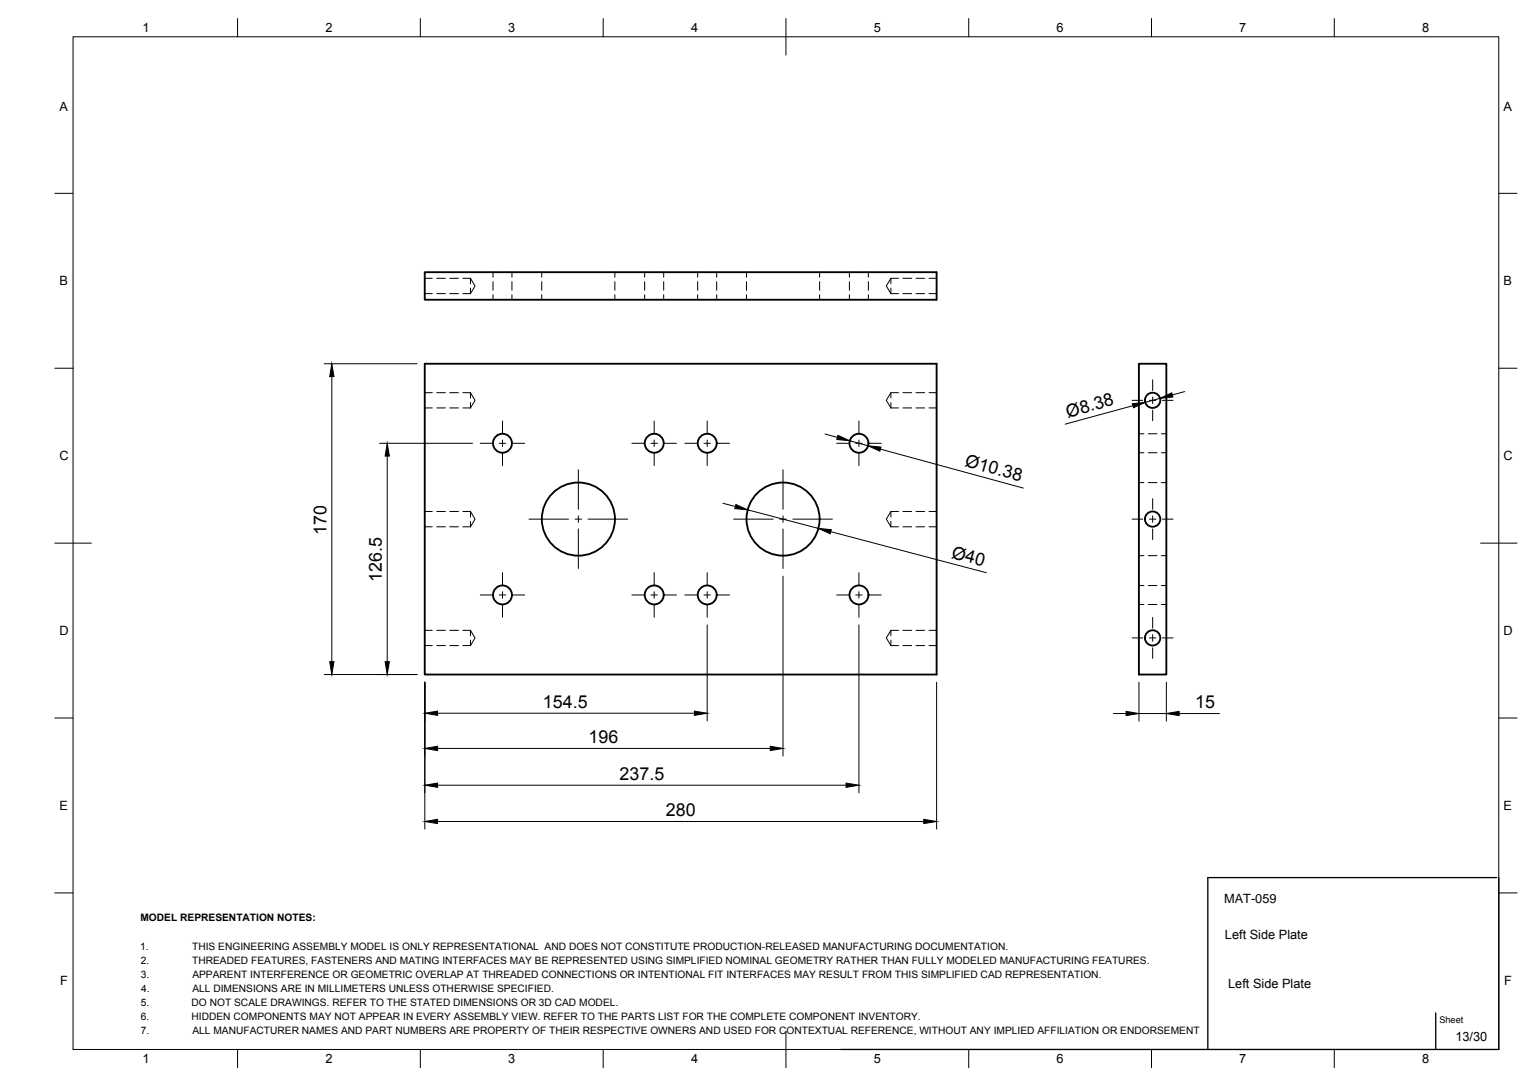
ISO-10303-21;
HEADER;
/* Generated by software containing ST-Developer
 * from STEP Tools, Inc. (www.steptools.com) 
 */

FILE_DESCRIPTION(
/* description */ ('', 'CAx-IF Rec.Pracs.---Representation and Presentation of Product Manufa
cturing Information (PMI)---4.0---2014-10-13'),
/* implementation_level */ '2;1');

FILE_NAME(
/* name */ 'Left Side Plate.step',
/* time_stamp */ '2026-10-28T23:00:48+01:00',
/* author */ (''),
/* organization */ (''),
/* preprocessor_version */ 'ST-DEVELOPER v20.2',
/* originating_system */ 'Autodesk Translation Framework v15.17.0.0',
/* authorisation */ '');

FILE_SCHEMA (('AP242_MANAGED_MODEL_BASED_3D_ENGINEERING_MIM_LF { 1 0 10303 442 2 1 4 }'));
ENDSEC;

DATA;
#10=MECHANICAL_DESIGN_GEOMETRIC_PRESENTATION_REPRESENTATION('',(#987),#61811);
#591=CONICAL_SURFACE('',#35772,2.094,1.02974425867665);
#592=CONICAL_SURFACE('',#35775,2.094,1.02974425867665);
#593=CONICAL_SURFACE('',#35778,2.094,1.02974425867665);
#594=CONICAL_SURFACE('',#35781,2.094,1.02974425867665);
#595=CONICAL_SURFACE('',#35784,2.094,1.02974425867665);
#596=CONICAL_SURFACE('',#35787,2.094,1.02974425867665);
#923=SHAPE_REPRESENTATION_RELATIONSHIP('SRR','None',#61982,#948);
#948=ADVANCED_BREP_SHAPE_REPRESENTATION('',(#1026),#61795);
#987=STYLED_ITEM('',(#62142),#1026);
#1026=MANIFOLD_SOLID_BREP('Body1',#33817);
#1327=CYLINDRICAL_SURFACE('',#35774,4.188);
#1328=CYLINDRICAL_SURFACE('',#35777,4.188);
#1329=CYLINDRICAL_SURFACE('',#35780,4.188);
#1330=CYLINDRICAL_SURFACE('',#35783,4.188);
#1331=CYLINDRICAL_SURFACE('',#35786,4.188);
#1332=CYLINDRICAL_SURFACE('',#35789,4.188);
#1333=CYLINDRICAL_SURFACE('',#35790,5.188);
#1334=CYLINDRICAL_SURFACE('',#35793,5.188);
#1335=CYLINDRICAL_SURFACE('',#35796,5.188);
#1336=CYLINDRICAL_SURFACE('',#35799,5.188);
#1337=CYLINDRICAL_SURFACE('',#35802,5.188);
#1338=CYLINDRICAL_SURFACE('',#35805,5.188);
#1339=CYLINDRICAL_SURFACE('',#35808,5.188);
#1340=CYLINDRICAL_SURFACE('',#35811,5.188);
#1341=CYLINDRICAL_SURFACE('',#35814,20.);
#1342=CYLINDRICAL_SURFACE('',#35817,20.);
#2042=FACE_BOUND('',#7145,.T.);
#2043=FACE_BOUND('',#7146,.T.);
#2044=FACE_BOUND('',#7147,.T.);
#2045=FACE_BOUND('',#7149,.T.);
#2046=FACE_BOUND('',#7150,.T.);
#2047=FACE_BOUND('',#7151,.T.);
#2048=FACE_BOUND('',#7176,.T.);
#2049=FACE_BOUND('',#7177,.T.);
#2050=FACE_BOUND('',#7178,.T.);
#2051=FACE_BOUND('',#7179,.T.);
#2052=FACE_BOUND('',#7180,.T.);
#2053=FACE_BOUND('',#7181,.T.);
#2054=FACE_BOUND('',#7182,.T.);
#2055=FACE_BOUND('',#7183,.T.);
#2056=FACE_BOUND('',#7184,.T.);
#2057=FACE_BOUND('',#7185,.T.);
#2058=FACE_BOUND('',#7188,.T.);
#2059=FACE_BOUND('',#7189,.T.);
#2060=FACE_BOUND('',#7190,.T.);
#2061=FACE_BOUND('',#7191,.T.);
#2062=FACE_BOUND('',#7192,.T.);
#2063=FACE_BOUND('',#7193,.T.);
#2064=FACE_BOUND('',#7194,.T.);
#2065=FACE_BOUND('',#7195,.T.);
#2066=FACE_BOUND('',#7196,.T.);
#2067=FACE_BOUND('',#7197,.T.);
#2952=CIRCLE('',#35764,4.188);
#2953=CIRCLE('',#35765,4.188);
#2954=CIRCLE('',#35766,4.188);
#2955=CIRCLE('',#35768,4.188);
#2956=CIRCLE('',#35769,4.188);
#2957=CIRCLE('',#35770,4.188);
#2958=CIRCLE('',#35773,4.188);
#2959=CIRCLE('',#35776,4.188);
#2960=CIRCLE('',#35779,4.188);
#2961=CIRCLE('',#35782,4.188);
#2962=CIRCLE('',#35785,4.188);
#2963=CIRCLE('',#35788,4.188);
#2964=CIRCLE('',#35791,5.188);
#2965=CIRCLE('',#35792,5.188);
#2966=CIRCLE('',#35794,5.188);
#2967=CIRCLE('',#35795,5.188);
#2968=CIRCLE('',#35797,5.188);
#2969=CIRCLE('',#35798,5.188);
#2970=CIRCLE('',#35800,5.188);
#2971=CIRCLE('',#35801,5.188);
#2972=CIRCLE('',#35803,5.188);
#2973=CIRCLE('',#35804,5.188);
#2974=CIRCLE('',#35806,5.188);
#2975=CIRCLE('',#35807,5.188);
#2976=CIRCLE('',#35809,5.188);
#2977=CIRCLE('',#35810,5.188);
#2978=CIRCLE('',#35812,5.188);
#2979=CIRCLE('',#35813,5.188);
#2980=CIRCLE('',#35815,20.);
#2981=CIRCLE('',#35816,20.);
#2982=CIRCLE('',#35818,20.);
#2983=CIRCLE('',#35819,20.);
#5102=FACE_OUTER_BOUND('',#7144,.T.);
#5103=FACE_OUTER_BOUND('',#7148,.T.);
#5104=FACE_OUTER_BOUND('',#7152,.T.);
#5105=FACE_OUTER_BOUND('',#7153,.T.);
#5106=FACE_OUTER_BOUND('',#7154,.T.);
#5107=FACE_OUTER_BOUND('',#7155,.T.);
#5108=FACE_OUTER_BOUND('',#7156,.T.);
#5109=FACE_OUTER_BOUND('',#7157,.T.);
#5110=FACE_OUTER_BOUND('',#7158,.T.);
#5111=FACE_OUTER_BOUND('',#7159,.T.);
#5112=FACE_OUTER_BOUND('',#7160,.T.);
#5113=FACE_OUTER_BOUND('',#7161,.T.);
#5114=FACE_OUTER_BOUND('',#7162,.T.);
#5115=FACE_OUTER_BOUND('',#7163,.T.);
#5116=FACE_OUTER_BOUND('',#7164,.T.);
#5117=FACE_OUTER_BOUND('',#7165,.T.);
#5118=FACE_OUTER_BOUND('',#7166,.T.);
#5119=FACE_OUTER_BOUND('',#7167,.T.);
#5120=FACE_OUTER_BOUND('',#7168,.T.);
#5121=FACE_OUTER_BOUND('',#7169,.T.);
#5122=FACE_OUTER_BOUND('',#7170,.T.);
#5123=FACE_OUTER_BOUND('',#7171,.T.);
#5124=FACE_OUTER_BOUND('',#7172,.T.);
#5125=FACE_OUTER_BOUND('',#7173,.T.);
#5126=FACE_OUTER_BOUND('',#7174,.T.);
#5127=FACE_OUTER_BOUND('',#7175,.T.);
#5128=FACE_OUTER_BOUND('',#7186,.T.);
#5129=FACE_OUTER_BOUND('',#7187,.T.);
#7144=EDGE_LOOP('',(#25798,#25799,#25800,#25801));
#7145=EDGE_LOOP('',(#25802));
#7146=EDGE_LOOP('',(#25803));
#7147=EDGE_LOOP('',(#25804));
#7148=EDGE_LOOP('',(#25805,#25806,#25807,#25808));
#7149=EDGE_LOOP('',(#25809));
#7150=EDGE_LOOP('',(#25810));
#7151=EDGE_LOOP('',(#25811));
#7152=EDGE_LOOP('',(#25812,#25813,#25814,#25815));
#7153=EDGE_LOOP('',(#25816,#25817,#25818));
#7154=EDGE_LOOP('',(#25819,#25820,#25821,#25822));
#7155=EDGE_LOOP('',(#25823,#25824,#25825));
#7156=EDGE_LOOP('',(#25826,#25827,#25828,#25829));
#7157=EDGE_LOOP('',(#25830,#25831,#25832));
#7158=EDGE_LOOP('',(#25833,#25834,#25835,#25836));
#7159=EDGE_LOOP('',(#25837,#25838,#25839));
#7160=EDGE_LOOP('',(#25840,#25841,#25842,#25843));
#7161=EDGE_LOOP('',(#25844,#25845,#25846));
#7162=EDGE_LOOP('',(#25847,#25848,#25849,#25850));
#7163=EDGE_LOOP('',(#25851,#25852,#25853));
#7164=EDGE_LOOP('',(#25854,#25855,#25856,#25857));
#7165=EDGE_LOOP('',(#25858,#25859,#25860,#25861));
#7166=EDGE_LOOP('',(#25862,#25863,#25864,#25865));
#7167=EDGE_LOOP('',(#25866,#25867,#25868,#25869));
#7168=EDGE_LOOP('',(#25870,#25871,#25872,#25873));
#7169=EDGE_LOOP('',(#25874,#25875,#25876,#25877));
#7170=EDGE_LOOP('',(#25878,#25879,#25880,#25881));
#7171=EDGE_LOOP('',(#25882,#25883,#25884,#25885));
#7172=EDGE_LOOP('',(#25886,#25887,#25888,#25889));
#7173=EDGE_LOOP('',(#25890,#25891,#25892,#25893));
#7174=EDGE_LOOP('',(#25894,#25895,#25896,#25897));
#7175=EDGE_LOOP('',(#25898,#25899,#25900,#25901));
#7176=EDGE_LOOP('',(#25902));
#7177=EDGE_LOOP('',(#25903));
#7178=EDGE_LOOP('',(#25904));
#7179=EDGE_LOOP('',(#25905));
#7180=EDGE_LOOP('',(#25906));
#7181=EDGE_LOOP('',(#25907));
#7182=EDGE_LOOP('',(#25908));
#7183=EDGE_LOOP('',(#25909));
#7184=EDGE_LOOP('',(#25910));
#7185=EDGE_LOOP('',(#25911));
#7186=EDGE_LOOP('',(#25912,#25913,#25914,#25915));
#7187=EDGE_LOOP('',(#25916,#25917,#25918,#25919));
#7188=EDGE_LOOP('',(#25920));
#7189=EDGE_LOOP('',(#25921));
#7190=EDGE_LOOP('',(#25922));
#7191=EDGE_LOOP('',(#25923));
#7192=EDGE_LOOP('',(#25924));
#7193=EDGE_LOOP('',(#25925));
#7194=EDGE_LOOP('',(#25926));
#7195=EDGE_LOOP('',(#25927));
#7196=EDGE_LOOP('',(#25928));
#7197=EDGE_LOOP('',(#25929));
#9621=LINE('',#55404,#12168);
#9622=LINE('',#55406,#12169);
#9623=LINE('',#55408,#12170);
#9624=LINE('',#55409,#12171);
#9625=LINE('',#55419,#12172);
#9626=LINE('',#55421,#12173);
#9627=LINE('',#55423,#12174);
#9628=LINE('',#55424,#12175);
#9629=LINE('',#55432,#12176);
#9630=LINE('',#55433,#12177);
#9631=LINE('',#55437,#12178);
#9632=LINE('',#55440,#12179);
#9633=LINE('',#55444,#12180);
#9634=LINE('',#55447,#12181);
#9635=LINE('',#55451,#12182);
#9636=LINE('',#55454,#12183);
#9637=LINE('',#55458,#12184);
#9638=LINE('',#55461,#12185);
#9639=LINE('',#55465,#12186);
#9640=LINE('',#55468,#12187);
#9641=LINE('',#55472,#12188);
#9642=LINE('',#55475,#12189);
#9643=LINE('',#55480,#12190);
#9644=LINE('',#55486,#12191);
#9645=LINE('',#55492,#12192);
#9646=LINE('',#55498,#12193);
#9647=LINE('',#55504,#12194);
#9648=LINE('',#55510,#12195);
#9649=LINE('',#55516,#12196);
#9650=LINE('',#55522,#12197);
#9651=LINE('',#55528,#12198);
#9652=LINE('',#55534,#12199);
#9653=LINE('',#55537,#12200);
#9654=LINE('',#55539,#12201);
#12168=VECTOR('',#42745,10.);
#12169=VECTOR('',#42746,10.);
#12170=VECTOR('',#42747,10.);
#12171=VECTOR('',#42748,10.);
#12172=VECTOR('',#42757,10.);
#12173=VECTOR('',#42758,10.);
#12174=VECTOR('',#42759,10.);
#12175=VECTOR('',#42760,10.);
#12176=VECTOR('',#42769,10.);
#12177=VECTOR('',#42770,10.);
#12178=VECTOR('',#42773,2.094);
#12179=VECTOR('',#42778,4.188);
#12180=VECTOR('',#42781,2.094);
#12181=VECTOR('',#42786,4.188);
#12182=VECTOR('',#42789,2.094);
#12183=VECTOR('',#42794,4.188);
#12184=VECTOR('',#42797,2.094);
#12185=VECTOR('',#42802,4.188);
#12186=VECTOR('',#42805,2.094);
#12187=VECTOR('',#42810,4.188);
#12188=VECTOR('',#42813,2.094);
#12189=VECTOR('',#42818,4.188);
#12190=VECTOR('',#42823,5.188);
#12191=VECTOR('',#42830,5.188);
#12192=VECTOR('',#42837,5.188);
#12193=VECTOR('',#42844,5.188);
#12194=VECTOR('',#42851,5.188);
#12195=VECTOR('',#42858,5.188);
#12196=VECTOR('',#42865,5.188);
#12197=VECTOR('',#42872,5.188);
#12198=VECTOR('',#42879,20.);
#12199=VECTOR('',#42886,20.);
#12200=VECTOR('',#42891,10.);
#12201=VECTOR('',#42894,10.);
#14850=VERTEX_POINT('',#55402);
#14851=VERTEX_POINT('',#55403);
#14852=VERTEX_POINT('',#55405);
#14853=VERTEX_POINT('',#55407);
#14854=VERTEX_POINT('',#55410);
#14855=VERTEX_POINT('',#55412);
#14856=VERTEX_POINT('',#55414);
#14857=VERTEX_POINT('',#55417);
#14858=VERTEX_POINT('',#55418);
#14859=VERTEX_POINT('',#55420);
#14860=VERTEX_POINT('',#55422);
#14861=VERTEX_POINT('',#55425);
#14862=VERTEX_POINT('',#55427);
#14863=VERTEX_POINT('',#55429);
#14864=VERTEX_POINT('',#55435);
#14865=VERTEX_POINT('',#55436);
#14866=VERTEX_POINT('',#55442);
#14867=VERTEX_POINT('',#55443);
#14868=VERTEX_POINT('',#55449);
#14869=VERTEX_POINT('',#55450);
#14870=VERTEX_POINT('',#55456);
#14871=VERTEX_POINT('',#55457);
#14872=VERTEX_POINT('',#55463);
#14873=VERTEX_POINT('',#55464);
#14874=VERTEX_POINT('',#55470);
#14875=VERTEX_POINT('',#55471);
#14876=VERTEX_POINT('',#55477);
#14877=VERTEX_POINT('',#55479);
#14878=VERTEX_POINT('',#55483);
#14879=VERTEX_POINT('',#55485);
#14880=VERTEX_POINT('',#55489);
#14881=VERTEX_POINT('',#55491);
#14882=VERTEX_POINT('',#55495);
#14883=VERTEX_POINT('',#55497);
#14884=VERTEX_POINT('',#55501);
#14885=VERTEX_POINT('',#55503);
#14886=VERTEX_POINT('',#55507);
#14887=VERTEX_POINT('',#55509);
#14888=VERTEX_POINT('',#55513);
#14889=VERTEX_POINT('',#55515);
#14890=VERTEX_POINT('',#55519);
#14891=VERTEX_POINT('',#55521);
#14892=VERTEX_POINT('',#55525);
#14893=VERTEX_POINT('',#55527);
#14894=VERTEX_POINT('',#55531);
#14895=VERTEX_POINT('',#55533);
#18801=EDGE_CURVE('',#14850,#14851,#9621,.T.);
#18802=EDGE_CURVE('',#14852,#14850,#9622,.T.);
#18803=EDGE_CURVE('',#14853,#14852,#9623,.T.);
#18804=EDGE_CURVE('',#14851,#14853,#9624,.T.);
#18805=EDGE_CURVE('',#14854,#14854,#2952,.T.);
#18806=EDGE_CURVE('',#14855,#14855,#2953,.T.);
#18807=EDGE_CURVE('',#14856,#14856,#2954,.T.);
#18808=EDGE_CURVE('',#14857,#14858,#9625,.T.);
#18809=EDGE_CURVE('',#14859,#14857,#9626,.T.);
#18810=EDGE_CURVE('',#14860,#14859,#9627,.T.);
#18811=EDGE_CURVE('',#14858,#14860,#9628,.T.);
#18812=EDGE_CURVE('',#14861,#14861,#2955,.T.);
#18813=EDGE_CURVE('',#14862,#14862,#2956,.T.);
#18814=EDGE_CURVE('',#14863,#14863,#2957,.T.);
#18815=EDGE_CURVE('',#14858,#14850,#9629,.T.);
#18816=EDGE_CURVE('',#14852,#14860,#9630,.T.);
#18817=EDGE_CURVE('',#14864,#14865,#9631,.T.);
#18818=EDGE_CURVE('',#14865,#14865,#2958,.T.);
#18819=EDGE_CURVE('',#14861,#14865,#9632,.T.);
#18820=EDGE_CURVE('',#14866,#14867,#9633,.T.);
#18821=EDGE_CURVE('',#14867,#14867,#2959,.T.);
#18822=EDGE_CURVE('',#14862,#14867,#9634,.T.);
#18823=EDGE_CURVE('',#14868,#14869,#9635,.T.);
#18824=EDGE_CURVE('',#14869,#14869,#2960,.T.);
#18825=EDGE_CURVE('',#14863,#14869,#9636,.T.);
#18826=EDGE_CURVE('',#14870,#14871,#9637,.T.);
#18827=EDGE_CURVE('',#14871,#14871,#2961,.T.);
#18828=EDGE_CURVE('',#14871,#14854,#9638,.T.);
#18829=EDGE_CURVE('',#14872,#14873,#9639,.T.);
#18830=EDGE_CURVE('',#14873,#14873,#2962,.T.);
#18831=EDGE_CURVE('',#14873,#14855,#9640,.T.);
#18832=EDGE_CURVE('',#14874,#14875,#9641,.T.);
#18833=EDGE_CURVE('',#14875,#14875,#2963,.T.);
#18834=EDGE_CURVE('',#14875,#14856,#9642,.T.);
#18835=EDGE_CURVE('',#14876,#14876,#2964,.T.);
#18836=EDGE_CURVE('',#14876,#14877,#9643,.T.);
#18837=EDGE_CURVE('',#14877,#14877,#2965,.T.);
#18838=EDGE_CURVE('',#14878,#14878,#2966,.T.);
#18839=EDGE_CURVE('',#14878,#14879,#9644,.T.);
#18840=EDGE_CURVE('',#14879,#14879,#2967,.T.);
#18841=EDGE_CURVE('',#14880,#14880,#2968,.T.);
#18842=EDGE_CURVE('',#14880,#14881,#9645,.T.);
#18843=EDGE_CURVE('',#14881,#14881,#2969,.T.);
#18844=EDGE_CURVE('',#14882,#14882,#2970,.T.);
#18845=EDGE_CURVE('',#14882,#14883,#9646,.T.);
#18846=EDGE_CURVE('',#14883,#14883,#2971,.T.);
#18847=EDGE_CURVE('',#14884,#14884,#2972,.T.);
#18848=EDGE_CURVE('',#14884,#14885,#9647,.T.);
#18849=EDGE_CURVE('',#14885,#14885,#2973,.T.);
#18850=EDGE_CURVE('',#14886,#14886,#2974,.T.);
#18851=EDGE_CURVE('',#14886,#14887,#9648,.T.);
#18852=EDGE_CURVE('',#14887,#14887,#2975,.T.);
#18853=EDGE_CURVE('',#14888,#14888,#2976,.T.);
#18854=EDGE_CURVE('',#14888,#14889,#9649,.T.);
#18855=EDGE_CURVE('',#14889,#14889,#2977,.T.);
#18856=EDGE_CURVE('',#14890,#14890,#2978,.T.);
#18857=EDGE_CURVE('',#14890,#14891,#9650,.T.);
#18858=EDGE_CURVE('',#14891,#14891,#2979,.T.);
#18859=EDGE_CURVE('',#14892,#14892,#2980,.T.);
#18860=EDGE_CURVE('',#14892,#14893,#9651,.T.);
#18861=EDGE_CURVE('',#14893,#14893,#2981,.T.);
#18862=EDGE_CURVE('',#14894,#14894,#2982,.T.);
#18863=EDGE_CURVE('',#14894,#14895,#9652,.T.);
#18864=EDGE_CURVE('',#14895,#14895,#2983,.T.);
#18865=EDGE_CURVE('',#14851,#14857,#9653,.T.);
#18866=EDGE_CURVE('',#14859,#14853,#9654,.T.);
#25798=ORIENTED_EDGE('',*,*,#18801,.F.);
#25799=ORIENTED_EDGE('',*,*,#18802,.F.);
#25800=ORIENTED_EDGE('',*,*,#18803,.F.);
#25801=ORIENTED_EDGE('',*,*,#18804,.F.);
#25802=ORIENTED_EDGE('',*,*,#18805,.F.);
#25803=ORIENTED_EDGE('',*,*,#18806,.F.);
#25804=ORIENTED_EDGE('',*,*,#18807,.F.);
#25805=ORIENTED_EDGE('',*,*,#18808,.F.);
#25806=ORIENTED_EDGE('',*,*,#18809,.F.);
#25807=ORIENTED_EDGE('',*,*,#18810,.F.);
#25808=ORIENTED_EDGE('',*,*,#18811,.F.);
#25809=ORIENTED_EDGE('',*,*,#18812,.F.);
#25810=ORIENTED_EDGE('',*,*,#18813,.F.);
#25811=ORIENTED_EDGE('',*,*,#18814,.F.);
#25812=ORIENTED_EDGE('',*,*,#18802,.T.);
#25813=ORIENTED_EDGE('',*,*,#18815,.F.);
#25814=ORIENTED_EDGE('',*,*,#18811,.T.);
#25815=ORIENTED_EDGE('',*,*,#18816,.F.);
#25816=ORIENTED_EDGE('',*,*,#18817,.T.);
#25817=ORIENTED_EDGE('',*,*,#18818,.F.);
#25818=ORIENTED_EDGE('',*,*,#18817,.F.);
#25819=ORIENTED_EDGE('',*,*,#18812,.T.);
#25820=ORIENTED_EDGE('',*,*,#18819,.T.);
#25821=ORIENTED_EDGE('',*,*,#18818,.T.);
#25822=ORIENTED_EDGE('',*,*,#18819,.F.);
#25823=ORIENTED_EDGE('',*,*,#18820,.T.);
#25824=ORIENTED_EDGE('',*,*,#18821,.F.);
#25825=ORIENTED_EDGE('',*,*,#18820,.F.);
#25826=ORIENTED_EDGE('',*,*,#18813,.T.);
#25827=ORIENTED_EDGE('',*,*,#18822,.T.);
#25828=ORIENTED_EDGE('',*,*,#18821,.T.);
#25829=ORIENTED_EDGE('',*,*,#18822,.F.);
#25830=ORIENTED_EDGE('',*,*,#18823,.T.);
#25831=ORIENTED_EDGE('',*,*,#18824,.F.);
#25832=ORIENTED_EDGE('',*,*,#18823,.F.);
#25833=ORIENTED_EDGE('',*,*,#18814,.T.);
#25834=ORIENTED_EDGE('',*,*,#18825,.T.);
#25835=ORIENTED_EDGE('',*,*,#18824,.T.);
#25836=ORIENTED_EDGE('',*,*,#18825,.F.);
#25837=ORIENTED_EDGE('',*,*,#18826,.T.);
#25838=ORIENTED_EDGE('',*,*,#18827,.T.);
#25839=ORIENTED_EDGE('',*,*,#18826,.F.);
#25840=ORIENTED_EDGE('',*,*,#18827,.F.);
#25841=ORIENTED_EDGE('',*,*,#18828,.T.);
#25842=ORIENTED_EDGE('',*,*,#18805,.T.);
#25843=ORIENTED_EDGE('',*,*,#18828,.F.);
#25844=ORIENTED_EDGE('',*,*,#18829,.T.);
#25845=ORIENTED_EDGE('',*,*,#18830,.T.);
#25846=ORIENTED_EDGE('',*,*,#18829,.F.);
#25847=ORIENTED_EDGE('',*,*,#18830,.F.);
#25848=ORIENTED_EDGE('',*,*,#18831,.T.);
#25849=ORIENTED_EDGE('',*,*,#18806,.T.);
#25850=ORIENTED_EDGE('',*,*,#18831,.F.);
#25851=ORIENTED_EDGE('',*,*,#18832,.T.);
#25852=ORIENTED_EDGE('',*,*,#18833,.T.);
#25853=ORIENTED_EDGE('',*,*,#18832,.F.);
#25854=ORIENTED_EDGE('',*,*,#18833,.F.);
#25855=ORIENTED_EDGE('',*,*,#18834,.T.);
#25856=ORIENTED_EDGE('',*,*,#18807,.T.);
#25857=ORIENTED_EDGE('',*,*,#18834,.F.);
#25858=ORIENTED_EDGE('',*,*,#18835,.F.);
#25859=ORIENTED_EDGE('',*,*,#18836,.T.);
#25860=ORIENTED_EDGE('',*,*,#18837,.F.);
#25861=ORIENTED_EDGE('',*,*,#18836,.F.);
#25862=ORIENTED_EDGE('',*,*,#18838,.F.);
#25863=ORIENTED_EDGE('',*,*,#18839,.T.);
#25864=ORIENTED_EDGE('',*,*,#18840,.F.);
#25865=ORIENTED_EDGE('',*,*,#18839,.F.);
#25866=ORIENTED_EDGE('',*,*,#18841,.F.);
#25867=ORIENTED_EDGE('',*,*,#18842,.T.);
#25868=ORIENTED_EDGE('',*,*,#18843,.F.);
#25869=ORIENTED_EDGE('',*,*,#18842,.F.);
#25870=ORIENTED_EDGE('',*,*,#18844,.F.);
#25871=ORIENTED_EDGE('',*,*,#18845,.T.);
#25872=ORIENTED_EDGE('',*,*,#18846,.F.);
#25873=ORIENTED_EDGE('',*,*,#18845,.F.);
#25874=ORIENTED_EDGE('',*,*,#18847,.F.);
#25875=ORIENTED_EDGE('',*,*,#18848,.T.);
#25876=ORIENTED_EDGE('',*,*,#18849,.F.);
#25877=ORIENTED_EDGE('',*,*,#18848,.F.);
#25878=ORIENTED_EDGE('',*,*,#18850,.F.);
#25879=ORIENTED_EDGE('',*,*,#18851,.T.);
#25880=ORIENTED_EDGE('',*,*,#18852,.F.);
#25881=ORIENTED_EDGE('',*,*,#18851,.F.);
#25882=ORIENTED_EDGE('',*,*,#18853,.F.);
#25883=ORIENTED_EDGE('',*,*,#18854,.T.);
#25884=ORIENTED_EDGE('',*,*,#18855,.F.);
#25885=ORIENTED_EDGE('',*,*,#18854,.F.);
#25886=ORIENTED_EDGE('',*,*,#18856,.F.);
#25887=ORIENTED_EDGE('',*,*,#18857,.T.);
#25888=ORIENTED_EDGE('',*,*,#18858,.F.);
#25889=ORIENTED_EDGE('',*,*,#18857,.F.);
#25890=ORIENTED_EDGE('',*,*,#18859,.F.);
#25891=ORIENTED_EDGE('',*,*,#18860,.T.);
#25892=ORIENTED_EDGE('',*,*,#18861,.F.);
#25893=ORIENTED_EDGE('',*,*,#18860,.F.);
#25894=ORIENTED_EDGE('',*,*,#18862,.F.);
#25895=ORIENTED_EDGE('',*,*,#18863,.T.);
#25896=ORIENTED_EDGE('',*,*,#18864,.F.);
#25897=ORIENTED_EDGE('',*,*,#18863,.F.);
#25898=ORIENTED_EDGE('',*,*,#18801,.T.);
#25899=ORIENTED_EDGE('',*,*,#18865,.T.);
#25900=ORIENTED_EDGE('',*,*,#18808,.T.);
#25901=ORIENTED_EDGE('',*,*,#18815,.T.);
#25902=ORIENTED_EDGE('',*,*,#18837,.T.);
#25903=ORIENTED_EDGE('',*,*,#18840,.T.);
#25904=ORIENTED_EDGE('',*,*,#18843,.T.);
#25905=ORIENTED_EDGE('',*,*,#18846,.T.);
#25906=ORIENTED_EDGE('',*,*,#18849,.T.);
#25907=ORIENTED_EDGE('',*,*,#18852,.T.);
#25908=ORIENTED_EDGE('',*,*,#18855,.T.);
#25909=ORIENTED_EDGE('',*,*,#18858,.T.);
#25910=ORIENTED_EDGE('',*,*,#18859,.T.);
#25911=ORIENTED_EDGE('',*,*,#18862,.T.);
#25912=ORIENTED_EDGE('',*,*,#18804,.T.);
#25913=ORIENTED_EDGE('',*,*,#18866,.F.);
#25914=ORIENTED_EDGE('',*,*,#18809,.T.);
#25915=ORIENTED_EDGE('',*,*,#18865,.F.);
#25916=ORIENTED_EDGE('',*,*,#18803,.T.);
#25917=ORIENTED_EDGE('',*,*,#18816,.T.);
#25918=ORIENTED_EDGE('',*,*,#18810,.T.);
#25919=ORIENTED_EDGE('',*,*,#18866,.T.);
#25920=ORIENTED_EDGE('',*,*,#18835,.T.);
#25921=ORIENTED_EDGE('',*,*,#18838,.T.);
#25922=ORIENTED_EDGE('',*,*,#18841,.T.);
#25923=ORIENTED_EDGE('',*,*,#18844,.T.);
#25924=ORIENTED_EDGE('',*,*,#18847,.T.);
#25925=ORIENTED_EDGE('',*,*,#18850,.T.);
#25926=ORIENTED_EDGE('',*,*,#18853,.T.);
#25927=ORIENTED_EDGE('',*,*,#18856,.T.);
#25928=ORIENTED_EDGE('',*,*,#18861,.T.);
#25929=ORIENTED_EDGE('',*,*,#18864,.T.);
#31588=PLANE('',#35763);
#31589=PLANE('',#35767);
#31590=PLANE('',#35771);
#31591=PLANE('',#35820);
#31592=PLANE('',#35821);
#31593=PLANE('',#35822);
#32783=ADVANCED_FACE('',(#5102,#2042,#2043,#2044),#31588,.F.);
#32784=ADVANCED_FACE('',(#5103,#2045,#2046,#2047),#31589,.F.);
#32785=ADVANCED_FACE('',(#5104),#31590,.T.);
#32786=ADVANCED_FACE('',(#5105),#591,.F.);
#32787=ADVANCED_FACE('',(#5106),#1327,.F.);
#32788=ADVANCED_FACE('',(#5107),#592,.F.);
#32789=ADVANCED_FACE('',(#5108),#1328,.F.);
#32790=ADVANCED_FACE('',(#5109),#593,.F.);
#32791=ADVANCED_FACE('',(#5110),#1329,.F.);
#32792=ADVANCED_FACE('',(#5111),#594,.F.);
#32793=ADVANCED_FACE('',(#5112),#1330,.F.);
#32794=ADVANCED_FACE('',(#5113),#595,.F.);
#32795=ADVANCED_FACE('',(#5114),#1331,.F.);
#32796=ADVANCED_FACE('',(#5115),#596,.F.);
#32797=ADVANCED_FACE('',(#5116),#1332,.F.);
#32798=ADVANCED_FACE('',(#5117),#1333,.F.);
#32799=ADVANCED_FACE('',(#5118),#1334,.F.);
#32800=ADVANCED_FACE('',(#5119),#1335,.F.);
#32801=ADVANCED_FACE('',(#5120),#1336,.F.);
#32802=ADVANCED_FACE('',(#5121),#1337,.F.);
#32803=ADVANCED_FACE('',(#5122),#1338,.F.);
#32804=ADVANCED_FACE('',(#5123),#1339,.F.);
#32805=ADVANCED_FACE('',(#5124),#1340,.F.);
#32806=ADVANCED_FACE('',(#5125),#1341,.F.);
#32807=ADVANCED_FACE('',(#5126),#1342,.F.);
#32808=ADVANCED_FACE('',(#5127,#2048,#2049,#2050,#2051,#2052,#2053,#2054,
#2055,#2056,#2057),#31591,.T.);
#32809=ADVANCED_FACE('',(#5128),#31592,.T.);
#32810=ADVANCED_FACE('',(#5129,#2058,#2059,#2060,#2061,#2062,#2063,#2064,
#2065,#2066,#2067),#31593,.T.);
#33817=CLOSED_SHELL('',(#32783,#32784,#32785,#32786,#32787,#32788,#32789,
#32790,#32791,#32792,#32793,#32794,#32795,#32796,#32797,#32798,#32799,#32800,
#32801,#32802,#32803,#32804,#32805,#32806,#32807,#32808,#32809,#32810));
#35762=AXIS2_PLACEMENT_3D('',#55400,#42741,#42742);
#35763=AXIS2_PLACEMENT_3D('',#55401,#42743,#42744);
#35764=AXIS2_PLACEMENT_3D('',#55411,#42749,#42750);
#35765=AXIS2_PLACEMENT_3D('',#55413,#42751,#42752);
#35766=AXIS2_PLACEMENT_3D('',#55415,#42753,#42754);
#35767=AXIS2_PLACEMENT_3D('',#55416,#42755,#42756);
#35768=AXIS2_PLACEMENT_3D('',#55426,#42761,#42762);
#35769=AXIS2_PLACEMENT_3D('',#55428,#42763,#42764);
#35770=AXIS2_PLACEMENT_3D('',#55430,#42765,#42766);
#35771=AXIS2_PLACEMENT_3D('',#55431,#42767,#42768);
#35772=AXIS2_PLACEMENT_3D('',#55434,#42771,#42772);
#35773=AXIS2_PLACEMENT_3D('',#55438,#42774,#42775);
#35774=AXIS2_PLACEMENT_3D('',#55439,#42776,#42777);
#35775=AXIS2_PLACEMENT_3D('',#55441,#42779,#42780);
#35776=AXIS2_PLACEMENT_3D('',#55445,#42782,#42783);
#35777=AXIS2_PLACEMENT_3D('',#55446,#42784,#42785);
#35778=AXIS2_PLACEMENT_3D('',#55448,#42787,#42788);
#35779=AXIS2_PLACEMENT_3D('',#55452,#42790,#42791);
#35780=AXIS2_PLACEMENT_3D('',#55453,#42792,#42793);
#35781=AXIS2_PLACEMENT_3D('',#55455,#42795,#42796);
#35782=AXIS2_PLACEMENT_3D('',#55459,#42798,#42799);
#35783=AXIS2_PLACEMENT_3D('',#55460,#42800,#42801);
#35784=AXIS2_PLACEMENT_3D('',#55462,#42803,#42804);
#35785=AXIS2_PLACEMENT_3D('',#55466,#42806,#42807);
#35786=AXIS2_PLACEMENT_3D('',#55467,#42808,#42809);
#35787=AXIS2_PLACEMENT_3D('',#55469,#42811,#42812);
#35788=AXIS2_PLACEMENT_3D('',#55473,#42814,#42815);
#35789=AXIS2_PLACEMENT_3D('',#55474,#42816,#42817);
#35790=AXIS2_PLACEMENT_3D('',#55476,#42819,#42820);
#35791=AXIS2_PLACEMENT_3D('',#55478,#42821,#42822);
#35792=AXIS2_PLACEMENT_3D('',#55481,#42824,#42825);
#35793=AXIS2_PLACEMENT_3D('',#55482,#42826,#42827);
#35794=AXIS2_PLACEMENT_3D('',#55484,#42828,#42829);
#35795=AXIS2_PLACEMENT_3D('',#55487,#42831,#42832);
#35796=AXIS2_PLACEMENT_3D('',#55488,#42833,#42834);
#35797=AXIS2_PLACEMENT_3D('',#55490,#42835,#42836);
#35798=AXIS2_PLACEMENT_3D('',#55493,#42838,#42839);
#35799=AXIS2_PLACEMENT_3D('',#55494,#42840,#42841);
#35800=AXIS2_PLACEMENT_3D('',#55496,#42842,#42843);
#35801=AXIS2_PLACEMENT_3D('',#55499,#42845,#42846);
#35802=AXIS2_PLACEMENT_3D('',#55500,#42847,#42848);
#35803=AXIS2_PLACEMENT_3D('',#55502,#42849,#42850);
#35804=AXIS2_PLACEMENT_3D('',#55505,#42852,#42853);
#35805=AXIS2_PLACEMENT_3D('',#55506,#42854,#42855);
#35806=AXIS2_PLACEMENT_3D('',#55508,#42856,#42857);
#35807=AXIS2_PLACEMENT_3D('',#55511,#42859,#42860);
#35808=AXIS2_PLACEMENT_3D('',#55512,#42861,#42862);
#35809=AXIS2_PLACEMENT_3D('',#55514,#42863,#42864);
#35810=AXIS2_PLACEMENT_3D('',#55517,#42866,#42867);
#35811=AXIS2_PLACEMENT_3D('',#55518,#42868,#42869);
#35812=AXIS2_PLACEMENT_3D('',#55520,#42870,#42871);
#35813=AXIS2_PLACEMENT_3D('',#55523,#42873,#42874);
#35814=AXIS2_PLACEMENT_3D('',#55524,#42875,#42876);
#35815=AXIS2_PLACEMENT_3D('',#55526,#42877,#42878);
#35816=AXIS2_PLACEMENT_3D('',#55529,#42880,#42881);
#35817=AXIS2_PLACEMENT_3D('',#55530,#42882,#42883);
#35818=AXIS2_PLACEMENT_3D('',#55532,#42884,#42885);
#35819=AXIS2_PLACEMENT_3D('',#55535,#42887,#42888);
#35820=AXIS2_PLACEMENT_3D('',#55536,#42889,#42890);
#35821=AXIS2_PLACEMENT_3D('',#55538,#42892,#42893);
#35822=AXIS2_PLACEMENT_3D('',#55540,#42895,#42896);
#42741=DIRECTION('axis',(0.,0.,1.));
#42742=DIRECTION('refdir',(1.,0.,0.));
#42743=DIRECTION('center_axis',(1.,-5.00596043934459E-16,-4.24079044878475E-15));
#42744=DIRECTION('ref_axis',(4.24079044878475E-15,-3.31747701864093E-15,
1.));
#42745=DIRECTION('',(-4.24079044878475E-15,3.31747701864093E-15,-1.));
#42746=DIRECTION('',(-5.00596043934473E-16,-1.,-3.31747701864093E-15));
#42747=DIRECTION('',(4.24079044878475E-15,-3.31747701864093E-15,1.));
#42748=DIRECTION('',(5.00596043934473E-16,1.,3.31747701864093E-15));
#42749=DIRECTION('center_axis',(-1.,5.00596043934459E-16,4.24079044878475E-15));
#42750=DIRECTION('ref_axis',(-5.00596043934473E-16,-1.,-3.31747701864093E-15));
#42751=DIRECTION('center_axis',(-1.,5.00596043934459E-16,4.24079044878475E-15));
#42752=DIRECTION('ref_axis',(-5.00596043934473E-16,-1.,-3.31747701864093E-15));
#42753=DIRECTION('center_axis',(-1.,5.00596043934459E-16,4.24079044878475E-15));
#42754=DIRECTION('ref_axis',(-5.00596043934473E-16,-1.,-3.31747701864093E-15));
#42755=DIRECTION('center_axis',(-1.,5.0059604393446E-16,3.87506992302587E-15));
#42756=DIRECTION('ref_axis',(-3.87506992302587E-15,3.31747701864093E-15,
-1.));
#42757=DIRECTION('',(3.87506992302587E-15,-3.31747701864093E-15,1.));
#42758=DIRECTION('',(-5.00596043934473E-16,-1.,-3.31747701864093E-15));
#42759=DIRECTION('',(-3.87506992302587E-15,3.31747701864093E-15,-1.));
#42760=DIRECTION('',(5.00596043934473E-16,1.,3.31747701864093E-15));
#42761=DIRECTION('center_axis',(1.,-5.0059604393446E-16,-3.87506992302587E-15));
#42762=DIRECTION('ref_axis',(-5.00596043934473E-16,-1.,-3.31747701864093E-15));
#42763=DIRECTION('center_axis',(1.,-5.0059604393446E-16,-3.87506992302587E-15));
#42764=DIRECTION('ref_axis',(-5.00596043934473E-16,-1.,-3.31747701864093E-15));
#42765=DIRECTION('center_axis',(1.,-5.0059604393446E-16,-3.87506992302587E-15));
#42766=DIRECTION('ref_axis',(-5.00596043934473E-16,-1.,-3.31747701864093E-15));
#42767=DIRECTION('center_axis',(3.82282413363175E-15,-3.31747701864093E-15,
1.));
#42768=DIRECTION('ref_axis',(1.,-5.00596043934461E-16,-3.82282413363175E-15));
#42769=DIRECTION('',(-1.,5.0059604393446E-16,3.82282413363175E-15));
#42770=DIRECTION('',(1.,-5.0059604393446E-16,-3.82282413363175E-15));
#42771=DIRECTION('center_axis',(1.,-5.0059604393446E-16,-3.82282413363175E-15));
#42772=DIRECTION('ref_axis',(-5.00596043934473E-16,-1.,-3.31747701864093E-15));
#42773=DIRECTION('',(0.515038074910054,0.857167300702112,9.79705557818207E-16));
#42774=DIRECTION('center_axis',(-1.,5.0059604393446E-16,3.82282413363175E-15));
#42775=DIRECTION('ref_axis',(-5.00596043934473E-16,-1.,-3.31747701864093E-15));
#42776=DIRECTION('center_axis',(-1.,5.0059604393446E-16,3.82282413363175E-15));
#42777=DIRECTION('ref_axis',(-5.00596043934473E-16,-1.,-3.31747701864093E-15));
#42778=DIRECTION('',(-1.,5.0059604393446E-16,3.82282413363175E-15));
#42779=DIRECTION('center_axis',(1.,-5.0059604393446E-16,-3.82282413363175E-15));
#42780=DIRECTION('ref_axis',(-5.00596043934473E-16,-1.,-3.31747701864093E-15));
#42781=DIRECTION('',(0.515038074910054,0.857167300702112,9.79705557818207E-16));
#42782=DIRECTION('center_axis',(-1.,5.0059604393446E-16,3.82282413363175E-15));
#42783=DIRECTION('ref_axis',(-5.00596043934473E-16,-1.,-3.31747701864093E-15));
#42784=DIRECTION('center_axis',(-1.,5.0059604393446E-16,3.82282413363175E-15));
#42785=DIRECTION('ref_axis',(-5.00596043934473E-16,-1.,-3.31747701864093E-15));
#42786=DIRECTION('',(-1.,5.0059604393446E-16,3.82282413363175E-15));
#42787=DIRECTION('center_axis',(1.,-5.0059604393446E-16,-3.82282413363175E-15));
#42788=DIRECTION('ref_axis',(-5.00596043934473E-16,-1.,-3.31747701864093E-15));
#42789=DIRECTION('',(0.515038074910054,0.857167300702112,9.79705557818207E-16));
#42790=DIRECTION('center_axis',(-1.,5.0059604393446E-16,3.82282413363175E-15));
#42791=DIRECTION('ref_axis',(-5.00596043934473E-16,-1.,-3.31747701864093E-15));
#42792=DIRECTION('center_axis',(-1.,5.0059604393446E-16,3.82282413363175E-15));
#42793=DIRECTION('ref_axis',(-5.00596043934473E-16,-1.,-3.31747701864093E-15));
#42794=DIRECTION('',(-1.,5.0059604393446E-16,3.82282413363175E-15));
#42795=DIRECTION('center_axis',(-1.,5.0059604393446E-16,3.82282413363175E-15));
#42796=DIRECTION('ref_axis',(-5.00596043934473E-16,-1.,-3.31747701864093E-15));
#42797=DIRECTION('',(-0.515038074910054,0.857167300702113,4.70756008460127E-15));
#42798=DIRECTION('center_axis',(-1.,5.0059604393446E-16,3.82282413363175E-15));
#42799=DIRECTION('ref_axis',(-5.00596043934473E-16,-1.,-3.31747701864093E-15));
#42800=DIRECTION('center_axis',(-1.,5.0059604393446E-16,3.82282413363175E-15));
#42801=DIRECTION('ref_axis',(-5.00596043934473E-16,-1.,-3.31747701864093E-15));
#42802=DIRECTION('',(-1.,5.0059604393446E-16,3.82282413363175E-15));
#42803=DIRECTION('center_axis',(-1.,5.0059604393446E-16,3.82282413363175E-15));
#42804=DIRECTION('ref_axis',(-5.00596043934473E-16,-1.,-3.31747701864093E-15));
#42805=DIRECTION('',(-0.515038074910054,0.857167300702113,4.70756008460127E-15));
#42806=DIRECTION('center_axis',(-1.,5.0059604393446E-16,3.82282413363175E-15));
#42807=DIRECTION('ref_axis',(-5.00596043934473E-16,-1.,-3.31747701864093E-15));
#42808=DIRECTION('center_axis',(-1.,5.0059604393446E-16,3.82282413363175E-15));
#42809=DIRECTION('ref_axis',(-5.00596043934473E-16,-1.,-3.31747701864093E-15));
#42810=DIRECTION('',(-1.,5.0059604393446E-16,3.82282413363175E-15));
#42811=DIRECTION('center_axis',(-1.,5.0059604393446E-16,3.82282413363175E-15));
#42812=DIRECTION('ref_axis',(-5.00596043934473E-16,-1.,-3.31747701864093E-15));
#42813=DIRECTION('',(-0.515038074910054,0.857167300702113,4.70756008460127E-15));
#42814=DIRECTION('center_axis',(-1.,5.0059604393446E-16,3.82282413363175E-15));
#42815=DIRECTION('ref_axis',(-5.00596043934473E-16,-1.,-3.31747701864093E-15));
#42816=DIRECTION('center_axis',(-1.,5.0059604393446E-16,3.82282413363175E-15));
#42817=DIRECTION('ref_axis',(-5.00596043934473E-16,-1.,-3.31747701864093E-15));
#42818=DIRECTION('',(-1.,5.0059604393446E-16,3.82282413363175E-15));
#42819=DIRECTION('center_axis',(-5.00596043934473E-16,-1.,-3.31747701864093E-15));
#42820=DIRECTION('ref_axis',(-1.,5.0059604393446E-16,3.82282413363175E-15));
#42821=DIRECTION('center_axis',(-5.00596043934473E-16,-1.,-3.31747701864093E-15));
#42822=DIRECTION('ref_axis',(-1.,5.0059604393446E-16,3.82282413363175E-15));
#42823=DIRECTION('',(-5.00596043934473E-16,-1.,-3.31747701864093E-15));
#42824=DIRECTION('center_axis',(5.00596043934473E-16,1.,3.31747701864093E-15));
#42825=DIRECTION('ref_axis',(-1.,5.0059604393446E-16,3.82282413363175E-15));
#42826=DIRECTION('center_axis',(-5.00596043934473E-16,-1.,-3.31747701864093E-15));
#42827=DIRECTION('ref_axis',(-1.,5.0059604393446E-16,3.82282413363175E-15));
#42828=DIRECTION('center_axis',(-5.00596043934473E-16,-1.,-3.31747701864093E-15));
#42829=DIRECTION('ref_axis',(-1.,5.0059604393446E-16,3.82282413363175E-15));
#42830=DIRECTION('',(-5.00596043934473E-16,-1.,-3.31747701864093E-15));
#42831=DIRECTION('center_axis',(5.00596043934473E-16,1.,3.31747701864093E-15));
#42832=DIRECTION('ref_axis',(-1.,5.0059604393446E-16,3.82282413363175E-15));
#42833=DIRECTION('center_axis',(-5.00596043934473E-16,-1.,-3.31747701864093E-15));
#42834=DIRECTION('ref_axis',(-1.,5.0059604393446E-16,3.82282413363175E-15));
#42835=DIRECTION('center_axis',(-5.00596043934473E-16,-1.,-3.31747701864093E-15));
#42836=DIRECTION('ref_axis',(-1.,5.0059604393446E-16,3.82282413363175E-15));
#42837=DIRECTION('',(-5.00596043934473E-16,-1.,-3.31747701864093E-15));
#42838=DIRECTION('center_axis',(5.00596043934473E-16,1.,3.31747701864093E-15));
#42839=DIRECTION('ref_axis',(-1.,5.0059604393446E-16,3.82282413363175E-15));
#42840=DIRECTION('center_axis',(-5.00596043934473E-16,-1.,-3.31747701864093E-15));
#42841=DIRECTION('ref_axis',(-1.,5.0059604393446E-16,3.82282413363175E-15));
#42842=DIRECTION('center_axis',(-5.00596043934473E-16,-1.,-3.31747701864093E-15));
#42843=DIRECTION('ref_axis',(-1.,5.0059604393446E-16,3.82282413363175E-15));
#42844=DIRECTION('',(-5.00596043934473E-16,-1.,-3.31747701864093E-15));
#42845=DIRECTION('center_axis',(5.00596043934473E-16,1.,3.31747701864093E-15));
#42846=DIRECTION('ref_axis',(-1.,5.0059604393446E-16,3.82282413363175E-15));
#42847=DIRECTION('center_axis',(-5.00596043934473E-16,-1.,-3.31747701864093E-15));
#42848=DIRECTION('ref_axis',(-1.,5.0059604393446E-16,3.82282413363175E-15));
#42849=DIRECTION('center_axis',(-5.00596043934473E-16,-1.,-3.31747701864093E-15));
#42850=DIRECTION('ref_axis',(-1.,5.0059604393446E-16,3.82282413363175E-15));
#42851=DIRECTION('',(-5.00596043934473E-16,-1.,-3.31747701864093E-15));
#42852=DIRECTION('center_axis',(5.00596043934473E-16,1.,3.31747701864093E-15));
#42853=DIRECTION('ref_axis',(-1.,5.0059604393446E-16,3.82282413363175E-15));
#42854=DIRECTION('center_axis',(-5.00596043934473E-16,-1.,-3.31747701864093E-15));
#42855=DIRECTION('ref_axis',(-1.,5.0059604393446E-16,3.82282413363175E-15));
#42856=DIRECTION('center_axis',(-5.00596043934473E-16,-1.,-3.31747701864093E-15));
#42857=DIRECTION('ref_axis',(-1.,5.0059604393446E-16,3.82282413363175E-15));
#42858=DIRECTION('',(-5.00596043934473E-16,-1.,-3.31747701864093E-15));
#42859=DIRECTION('center_axis',(5.00596043934473E-16,1.,3.31747701864093E-15));
#42860=DIRECTION('ref_axis',(-1.,5.0059604393446E-16,3.82282413363175E-15));
#42861=DIRECTION('center_axis',(-5.00596043934473E-16,-1.,-3.31747701864093E-15));
#42862=DIRECTION('ref_axis',(-1.,5.0059604393446E-16,3.82282413363175E-15));
#42863=DIRECTION('center_axis',(-5.00596043934473E-16,-1.,-3.31747701864093E-15));
#42864=DIRECTION('ref_axis',(-1.,5.0059604393446E-16,3.82282413363175E-15));
#42865=DIRECTION('',(-5.00596043934473E-16,-1.,-3.31747701864093E-15));
#42866=DIRECTION('center_axis',(5.00596043934473E-16,1.,3.31747701864093E-15));
#42867=DIRECTION('ref_axis',(-1.,5.0059604393446E-16,3.82282413363175E-15));
#42868=DIRECTION('center_axis',(-5.00596043934473E-16,-1.,-3.31747701864093E-15));
#42869=DIRECTION('ref_axis',(-1.,5.0059604393446E-16,3.82282413363175E-15));
#42870=DIRECTION('center_axis',(-5.00596043934473E-16,-1.,-3.31747701864093E-15));
#42871=DIRECTION('ref_axis',(-1.,5.0059604393446E-16,3.82282413363175E-15));
#42872=DIRECTION('',(-5.00596043934473E-16,-1.,-3.31747701864093E-15));
#42873=DIRECTION('center_axis',(5.00596043934473E-16,1.,3.31747701864093E-15));
#42874=DIRECTION('ref_axis',(-1.,5.0059604393446E-16,3.82282413363175E-15));
#42875=DIRECTION('center_axis',(5.00596043934473E-16,1.,3.31747701864093E-15));
#42876=DIRECTION('ref_axis',(1.,-5.0059604393446E-16,-3.82282413363175E-15));
#42877=DIRECTION('center_axis',(5.00596043934473E-16,1.,3.31747701864093E-15));
#42878=DIRECTION('ref_axis',(1.,-5.0059604393446E-16,-3.82282413363175E-15));
#42879=DIRECTION('',(5.00596043934473E-16,1.,3.31747701864093E-15));
#42880=DIRECTION('center_axis',(-5.00596043934473E-16,-1.,-3.31747701864093E-15));
#42881=DIRECTION('ref_axis',(1.,-5.0059604393446E-16,-3.82282413363175E-15));
#42882=DIRECTION('center_axis',(5.00596043934473E-16,1.,3.31747701864093E-15));
#42883=DIRECTION('ref_axis',(1.,-5.0059604393446E-16,-3.82282413363175E-15));
#42884=DIRECTION('center_axis',(5.00596043934473E-16,1.,3.31747701864093E-15));
#42885=DIRECTION('ref_axis',(1.,-5.0059604393446E-16,-3.82282413363175E-15));
#42886=DIRECTION('',(5.00596043934473E-16,1.,3.31747701864093E-15));
#42887=DIRECTION('center_axis',(-5.00596043934473E-16,-1.,-3.31747701864093E-15));
#42888=DIRECTION('ref_axis',(1.,-5.0059604393446E-16,-3.82282413363175E-15));
#42889=DIRECTION('center_axis',(-5.00596043934473E-16,-1.,-3.31747701864093E-15));
#42890=DIRECTION('ref_axis',(1.,-5.00596043934461E-16,-3.82282413363175E-15));
#42891=DIRECTION('',(1.,-5.0059604393446E-16,-3.82282413363175E-15));
#42892=DIRECTION('center_axis',(-3.82282413363175E-15,3.31747701864093E-15,
-1.));
#42893=DIRECTION('ref_axis',(-1.,5.00596043934461E-16,3.82282413363175E-15));
#42894=DIRECTION('',(-1.,5.0059604393446E-16,3.82282413363175E-15));
#42895=DIRECTION('center_axis',(5.00596043934473E-16,1.,3.31747701864093E-15));
#42896=DIRECTION('ref_axis',(-1.,5.00596043934461E-16,3.82282413363175E-15));
#55400=CARTESIAN_POINT('',(0.,0.,0.));
#55401=CARTESIAN_POINT('Origin',(179.115917770968,-85.4720072687897,360.000000551894));
#55402=CARTESIAN_POINT('',(179.115917770968,-100.47200726879,530.000000551894));
#55403=CARTESIAN_POINT('',(179.115917770968,-100.47200726879,360.000000551894));
#55404=CARTESIAN_POINT('',(179.115917770968,-100.47200726879,402.500000551894));
#55405=CARTESIAN_POINT('',(179.115917770968,-85.4720072687903,530.000000551894));
#55406=CARTESIAN_POINT('',(179.115917770968,-89.2220072687903,530.000000551894));
#55407=CARTESIAN_POINT('',(179.115917770968,-85.4720072687897,360.000000551894));
#55408=CARTESIAN_POINT('',(179.115917770968,-85.4720072687898,402.500000551894));
#55409=CARTESIAN_POINT('',(179.115917770968,-89.2220072687897,360.000000551894));
#55410=CARTESIAN_POINT('',(179.115917770968,-88.7840072687902,510.000000551894));
#55411=CARTESIAN_POINT('Origin',(179.115917770968,-92.9720072687902,510.000000551894));
#55412=CARTESIAN_POINT('',(179.115917770968,-88.7840072687899,445.000000551894));
#55413=CARTESIAN_POINT('Origin',(179.115917770968,-92.97200726879,445.000000551894));
#55414=CARTESIAN_POINT('',(179.115917770968,-88.7840072687897,380.000000551894));
#55415=CARTESIAN_POINT('Origin',(179.115917770968,-92.9720072687898,380.000000551894));
#55416=CARTESIAN_POINT('Origin',(459.115917770968,-85.4720072687904,530.000000551893));
#55417=CARTESIAN_POINT('',(459.115917770968,-100.47200726879,360.000000551893));
#55418=CARTESIAN_POINT('',(459.115917770968,-100.47200726879,530.000000551893));
#55419=CARTESIAN_POINT('',(459.115917770968,-100.47200726879,487.500000551893));
#55420=CARTESIAN_POINT('',(459.115917770968,-85.4720072687898,360.000000551893));
#55421=CARTESIAN_POINT('',(459.115917770968,-89.2220072687898,360.000000551893));
#55422=CARTESIAN_POINT('',(459.115917770968,-85.4720072687904,530.000000551893));
#55423=CARTESIAN_POINT('',(459.115917770968,-85.4720072687903,487.500000551893));
#55424=CARTESIAN_POINT('',(459.115917770968,-89.2220072687904,530.000000551893));
#55425=CARTESIAN_POINT('',(459.115917770968,-88.7840072687903,510.000000551893));
#55426=CARTESIAN_POINT('Origin',(459.115917770968,-92.9720072687903,510.000000551893));
#55427=CARTESIAN_POINT('',(459.115917770968,-88.7840072687901,445.000000551893));
#55428=CARTESIAN_POINT('Origin',(459.115917770968,-92.9720072687901,445.000000551893));
#55429=CARTESIAN_POINT('',(459.115917770968,-88.7840072687899,380.000000551893));
#55430=CARTESIAN_POINT('Origin',(459.115917770968,-92.9720072687899,380.000000551893));
#55431=CARTESIAN_POINT('Origin',(164.115917770968,-92.9720072687902,530.000000551894));
#55432=CARTESIAN_POINT('',(474.115917770968,-100.47200726879,530.000000551893));
#55433=CARTESIAN_POINT('',(474.115917770968,-85.4720072687904,530.000000551893));
#55434=CARTESIAN_POINT('Origin',(432.857715634724,-92.9720072687903,510.000000551893));
#55435=CARTESIAN_POINT('',(431.599513498481,-92.9720072687903,510.000000551893));
#55436=CARTESIAN_POINT('',(434.115917770968,-88.7840072687902,510.000000551893));
#55437=CARTESIAN_POINT('',(432.857715634724,-90.8780072687903,510.000000551893));
#55438=CARTESIAN_POINT('Origin',(434.115917770968,-92.9720072687903,510.000000551893));
#55439=CARTESIAN_POINT('Origin',(454.115917770968,-92.9720072687903,510.000000551893));
#55440=CARTESIAN_POINT('',(454.115917770968,-88.7840072687903,510.000000551893));
#55441=CARTESIAN_POINT('Origin',(432.857715634724,-92.9720072687901,445.000000551893));
#55442=CARTESIAN_POINT('',(431.599513498481,-92.9720072687901,445.000000551893));
#55443=CARTESIAN_POINT('',(434.115917770968,-88.78400726879,445.000000551893));
#55444=CARTESIAN_POINT('',(432.857715634724,-90.8780072687901,445.000000551893));
#55445=CARTESIAN_POINT('Origin',(434.115917770968,-92.9720072687901,445.000000551893));
#55446=CARTESIAN_POINT('Origin',(454.115917770968,-92.9720072687901,445.000000551893));
#55447=CARTESIAN_POINT('',(454.115917770968,-88.7840072687901,445.000000551893));
#55448=CARTESIAN_POINT('Origin',(432.857715634724,-92.9720072687899,380.000000551893));
#55449=CARTESIAN_POINT('',(431.59951349848,-92.9720072687899,380.000000551893));
#55450=CARTESIAN_POINT('',(434.115917770968,-88.7840072687898,380.000000551893));
#55451=CARTESIAN_POINT('',(432.857715634724,-90.8780072687899,380.000000551893));
#55452=CARTESIAN_POINT('Origin',(434.115917770968,-92.9720072687899,380.000000551893));
#55453=CARTESIAN_POINT('Origin',(454.115917770968,-92.9720072687899,380.000000551893));
#55454=CARTESIAN_POINT('',(454.115917770968,-88.7840072687899,380.000000551893));
#55455=CARTESIAN_POINT('Origin',(205.374119907212,-92.9720072687902,510.000000551894));
#55456=CARTESIAN_POINT('',(206.632322043456,-92.9720072687902,510.000000551894));
#55457=CARTESIAN_POINT('',(204.115917770968,-88.7840072687901,510.000000551894));
#55458=CARTESIAN_POINT('',(205.374119907212,-90.8780072687902,510.000000551894));
#55459=CARTESIAN_POINT('Origin',(204.115917770968,-92.9720072687902,510.000000551894));
#55460=CARTESIAN_POINT('Origin',(184.115917770968,-92.9720072687902,510.000000551894));
#55461=CARTESIAN_POINT('',(184.115917770968,-88.7840072687902,510.000000551894));
#55462=CARTESIAN_POINT('Origin',(205.374119907212,-92.97200726879,445.000000551894));
#55463=CARTESIAN_POINT('',(206.632322043456,-92.97200726879,445.000000551894));
#55464=CARTESIAN_POINT('',(204.115917770968,-88.7840072687898,445.000000551894));
#55465=CARTESIAN_POINT('',(205.374119907212,-90.87800726879,445.000000551894));
#55466=CARTESIAN_POINT('Origin',(204.115917770968,-92.97200726879,445.000000551894));
#55467=CARTESIAN_POINT('Origin',(184.115917770968,-92.97200726879,445.000000551894));
#55468=CARTESIAN_POINT('',(184.115917770968,-88.78400726879,445.000000551894));
#55469=CARTESIAN_POINT('Origin',(205.374119907212,-92.9720072687898,380.000000551894));
#55470=CARTESIAN_POINT('',(206.632322043455,-92.9720072687898,380.000000551894));
#55471=CARTESIAN_POINT('',(204.115917770968,-88.7840072687896,380.000000551894));
#55472=CARTESIAN_POINT('',(205.374119907212,-90.8780072687897,380.000000551894));
#55473=CARTESIAN_POINT('Origin',(204.115917770968,-92.9720072687898,380.000000551894));
#55474=CARTESIAN_POINT('Origin',(184.115917770968,-92.9720072687898,380.000000551894));
#55475=CARTESIAN_POINT('',(184.115917770968,-88.7840072687898,380.000000551894));
#55476=CARTESIAN_POINT('Origin',(221.615917770968,-84.8220072687901,486.500000551894));
#55477=CARTESIAN_POINT('',(226.803917770968,-85.4720072687901,486.500000551894));
#55478=CARTESIAN_POINT('Origin',(221.615917770968,-85.4720072687901,486.500000551894));
#55479=CARTESIAN_POINT('',(226.803917770968,-100.47200726879,486.500000551894));
#55480=CARTESIAN_POINT('',(226.803917770968,-84.8220072687901,486.500000551894));
#55481=CARTESIAN_POINT('Origin',(221.615917770968,-100.47200726879,486.500000551894));
#55482=CARTESIAN_POINT('Origin',(333.615917770968,-84.8220072687899,403.500000551893));
#55483=CARTESIAN_POINT('',(338.803917770968,-85.4720072687899,403.500000551893));
#55484=CARTESIAN_POINT('Origin',(333.615917770968,-85.4720072687899,403.500000551893));
#55485=CARTESIAN_POINT('',(338.803917770968,-100.47200726879,403.500000551893));
#55486=CARTESIAN_POINT('',(338.803917770968,-84.8220072687899,403.500000551893));
#55487=CARTESIAN_POINT('Origin',(333.615917770968,-100.47200726879,403.500000551893));
#55488=CARTESIAN_POINT('Origin',(333.615917770968,-84.8220072687902,486.500000551893));
#55489=CARTESIAN_POINT('',(338.803917770968,-85.4720072687902,486.500000551893));
#55490=CARTESIAN_POINT('Origin',(333.615917770968,-85.4720072687902,486.500000551893));
#55491=CARTESIAN_POINT('',(338.803917770968,-100.47200726879,486.500000551893));
#55492=CARTESIAN_POINT('',(338.803917770968,-84.8220072687902,486.500000551893));
#55493=CARTESIAN_POINT('Origin',(333.615917770968,-100.47200726879,486.500000551893));
#55494=CARTESIAN_POINT('Origin',(416.615917770968,-84.8220072687902,486.500000551893));
#55495=CARTESIAN_POINT('',(421.803917770968,-85.4720072687902,486.500000551893));
#55496=CARTESIAN_POINT('Origin',(416.615917770968,-85.4720072687902,486.500000551893));
#55497=CARTESIAN_POINT('',(421.803917770968,-100.47200726879,486.500000551893));
#55498=CARTESIAN_POINT('',(421.803917770968,-84.8220072687902,486.500000551893));
#55499=CARTESIAN_POINT('Origin',(416.615917770968,-100.47200726879,486.500000551893));
#55500=CARTESIAN_POINT('Origin',(416.615917770968,-84.8220072687899,403.500000551893));
#55501=CARTESIAN_POINT('',(421.803917770968,-85.47200726879,403.500000551893));
#55502=CARTESIAN_POINT('Origin',(416.615917770968,-85.47200726879,403.500000551893));
#55503=CARTESIAN_POINT('',(421.803917770968,-100.47200726879,403.500000551893));
#55504=CARTESIAN_POINT('',(421.803917770968,-84.8220072687899,403.500000551893));
#55505=CARTESIAN_POINT('Origin',(416.615917770968,-100.47200726879,403.500000551893));
#55506=CARTESIAN_POINT('Origin',(304.615917770968,-84.8220072687902,486.500000551893));
#55507=CARTESIAN_POINT('',(309.803917770968,-85.4720072687902,486.500000551893));
#55508=CARTESIAN_POINT('Origin',(304.615917770968,-85.4720072687902,486.500000551893));
#55509=CARTESIAN_POINT('',(309.803917770968,-100.47200726879,486.500000551893));
#55510=CARTESIAN_POINT('',(309.803917770968,-84.8220072687902,486.500000551893));
#55511=CARTESIAN_POINT('Origin',(304.615917770968,-100.47200726879,486.500000551893));
#55512=CARTESIAN_POINT('Origin',(304.615917770968,-84.8220072687899,403.500000551893));
#55513=CARTESIAN_POINT('',(309.803917770968,-85.4720072687899,403.500000551893));
#55514=CARTESIAN_POINT('Origin',(304.615917770968,-85.4720072687899,403.500000551893));
#55515=CARTESIAN_POINT('',(309.803917770968,-100.47200726879,403.500000551893));
#55516=CARTESIAN_POINT('',(309.803917770968,-84.8220072687899,403.500000551893));
#55517=CARTESIAN_POINT('Origin',(304.615917770968,-100.47200726879,403.500000551893));
#55518=CARTESIAN_POINT('Origin',(221.615917770968,-84.8220072687898,403.500000551894));
#55519=CARTESIAN_POINT('',(226.803917770968,-85.4720072687898,403.500000551894));
#55520=CARTESIAN_POINT('Origin',(221.615917770968,-85.4720072687898,403.500000551894));
#55521=CARTESIAN_POINT('',(226.803917770968,-100.47200726879,403.500000551893));
#55522=CARTESIAN_POINT('',(226.803917770968,-84.8220072687898,403.500000551894));
#55523=CARTESIAN_POINT('Origin',(221.615917770968,-100.47200726879,403.500000551894));
#55524=CARTESIAN_POINT('Origin',(375.115917770968,-100.47200726879,445.000000551893));
#55525=CARTESIAN_POINT('',(355.115917770968,-100.47200726879,445.000000551893));
#55526=CARTESIAN_POINT('Origin',(375.115917770968,-100.47200726879,445.000000551893));
#55527=CARTESIAN_POINT('',(355.115917770968,-85.4720072687901,445.000000551893));
#55528=CARTESIAN_POINT('',(355.115917770968,-100.47200726879,445.000000551893));
#55529=CARTESIAN_POINT('Origin',(375.115917770968,-85.4720072687901,445.000000551893));
#55530=CARTESIAN_POINT('Origin',(263.115917770968,-100.47200726879,445.000000551893));
#55531=CARTESIAN_POINT('',(243.115917770968,-100.47200726879,445.000000551893));
#55532=CARTESIAN_POINT('Origin',(263.115917770968,-100.47200726879,445.000000551893));
#55533=CARTESIAN_POINT('',(243.115917770968,-85.47200726879,445.000000551893));
#55534=CARTESIAN_POINT('',(243.115917770968,-100.47200726879,445.000000551893));
#55535=CARTESIAN_POINT('Origin',(263.115917770968,-85.47200726879,445.000000551893));
#55536=CARTESIAN_POINT('Origin',(319.115917770968,-100.47200726879,445.000000551893));
#55537=CARTESIAN_POINT('',(164.115917770968,-100.47200726879,360.000000551894));
#55538=CARTESIAN_POINT('Origin',(474.115917770968,-92.9720072687898,360.000000551893));
#55539=CARTESIAN_POINT('',(164.115917770968,-85.4720072687897,360.000000551894));
#55540=CARTESIAN_POINT('Origin',(319.115917770968,-85.47200726879,445.000000551893));
#61764=UNCERTAINTY_MEASURE_WITH_UNIT(LENGTH_MEASURE(0.01),#61812,
'DISTANCE_ACCURACY_VALUE',
'Maximum model space distance between geometric entities at asserted c
onnectivities');
#61780=UNCERTAINTY_MEASURE_WITH_UNIT(LENGTH_MEASURE(0.01),#61812,
'DISTANCE_ACCURACY_VALUE',
'Maximum model space distance between geometric entities at asserted c
onnectivities');
#61795=(
GEOMETRIC_REPRESENTATION_CONTEXT(3)
GLOBAL_UNCERTAINTY_ASSIGNED_CONTEXT((#61764))
GLOBAL_UNIT_ASSIGNED_CONTEXT((#61812,#61814,#61815))
REPRESENTATION_CONTEXT('','3D')
);
#61811=(
GEOMETRIC_REPRESENTATION_CONTEXT(3)
GLOBAL_UNCERTAINTY_ASSIGNED_CONTEXT((#61780))
GLOBAL_UNIT_ASSIGNED_CONTEXT((#61812,#61814,#61815))
REPRESENTATION_CONTEXT('','3D')
);
#61812=(
LENGTH_UNIT()
NAMED_UNIT(*)
SI_UNIT(.MILLI.,.METRE.)
);
#61814=(
NAMED_UNIT(*)
PLANE_ANGLE_UNIT()
SI_UNIT($,.RADIAN.)
);
#61815=(
NAMED_UNIT(*)
SI_UNIT($,.STERADIAN.)
SOLID_ANGLE_UNIT()
);
#61830=SHAPE_DEFINITION_REPRESENTATION(#61860,#61982);
#61860=PRODUCT_DEFINITION_SHAPE('',$,#62013);
#61982=SHAPE_REPRESENTATION('',(#35762),#61795);
#61998=PRODUCT_DEFINITION_CONTEXT('part definition',#62090,'design');
#62013=PRODUCT_DEFINITION('Left Side Plate','Left Side Plate',#62043,#61998);
#62043=PRODUCT_DEFINITION_FORMATION('',$,#62106);
#62090=APPLICATION_CONTEXT('Managed model based 3d engineering');
#62091=PRODUCT_CONTEXT('part definition',#62090,'mechanical');
#62106=PRODUCT('Left Side Plate','Left Side Plate',$,(#62091));
#62136=COLOUR_RGB('Light Blue',0.38,0.62,0.78);
#62137=FILL_AREA_STYLE_COLOUR('',#62136);
#62138=FILL_AREA_STYLE('',(#62137));
#62139=SURFACE_STYLE_FILL_AREA(#62138);
#62140=SURFACE_SIDE_STYLE('',(#62139));
#62141=SURFACE_STYLE_USAGE(.BOTH.,#62140);
#62142=PRESENTATION_STYLE_ASSIGNMENT((#62141));
ENDSEC;
END-ISO-10303-21;
